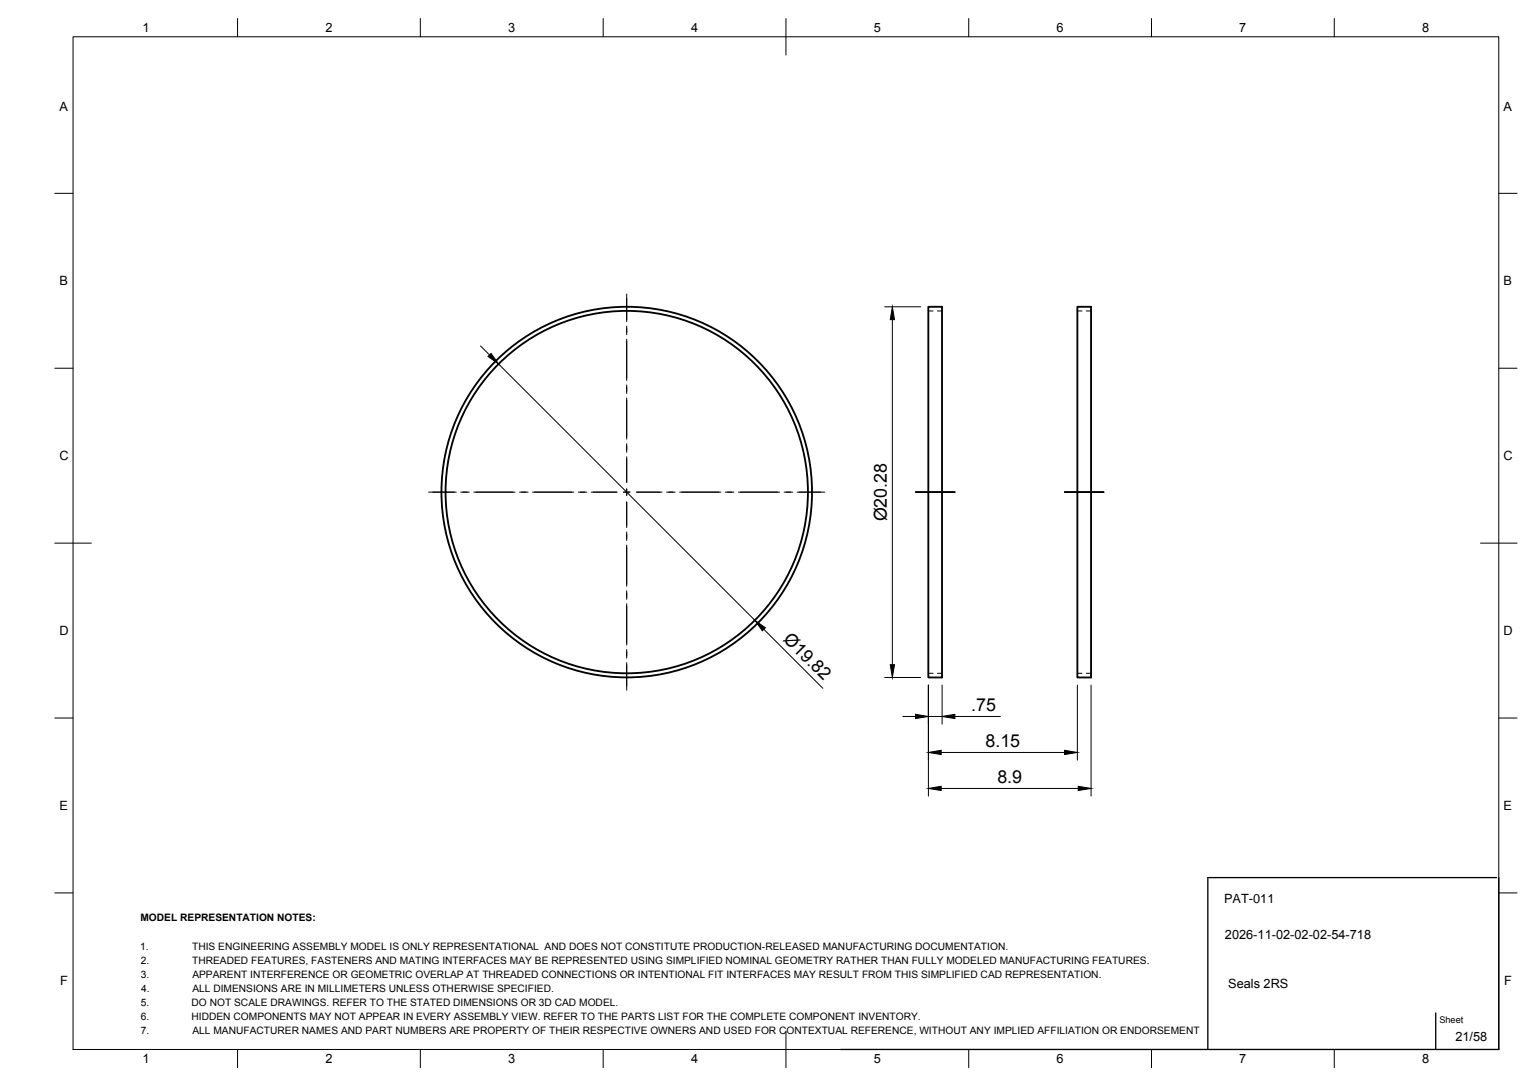
ISO-10303-21;
HEADER;
/* Generated by software containing ST-Developer
 * from STEP Tools, Inc. (www.steptools.com) 
 */

FILE_DESCRIPTION(
/* description */ ('Belt tension measurement rig'),
/* implementation_level */ '2;1');

FILE_NAME(
/* name */ 'Seals 2RS.step',
/* time_stamp */ '2026-10-28T03:24:44-07:00',
/* author */ (''),
/* organization */ (''),
/* preprocessor_version */ 'ST-DEVELOPER v20.2',
/* originating_system */ 'Autodesk Translation Framework v15.17.0.0',
/* authorisation */ '');

FILE_SCHEMA (('AUTOMOTIVE_DESIGN { 1 0 10303 214 3 1 1 }'));
ENDSEC;

DATA;
#10=MECHANICAL_DESIGN_GEOMETRIC_PRESENTATION_REPRESENTATION('',(#717,#718),#23587);
#600=SHAPE_REPRESENTATION_RELATIONSHIP('SRR','None',#23846,#655);
#655=ADVANCED_BREP_SHAPE_REPRESENTATION('',(#787,#788),#23544);
#717=STYLED_ITEM('',(#24211),#787);
#718=STYLED_ITEM('',(#24211),#788);
#787=MANIFOLD_SOLID_BREP('Body1',#12222);
#788=MANIFOLD_SOLID_BREP('Body2',#12223);
#912=FACE_BOUND('',#2360,.T.);
#913=FACE_BOUND('',#2363,.T.);
#914=FACE_BOUND('',#2366,.T.);
#915=FACE_BOUND('',#2369,.T.);
#1151=PLANE('',#13334);
#1152=PLANE('',#13339);
#1153=PLANE('',#13342);
#1154=PLANE('',#13347);
#1572=FACE_OUTER_BOUND('',#2359,.T.);
#1573=FACE_OUTER_BOUND('',#2361,.T.);
#1574=FACE_OUTER_BOUND('',#2362,.T.);
#1575=FACE_OUTER_BOUND('',#2364,.T.);
#1576=FACE_OUTER_BOUND('',#2365,.T.);
#1577=FACE_OUTER_BOUND('',#2367,.T.);
#1578=FACE_OUTER_BOUND('',#2368,.T.);
#1579=FACE_OUTER_BOUND('',#2370,.T.);
#2359=EDGE_LOOP('',(#8872));
#2360=EDGE_LOOP('',(#8873));
#2361=EDGE_LOOP('',(#8874,#8875,#8876,#8877));
#2362=EDGE_LOOP('',(#8878));
#2363=EDGE_LOOP('',(#8879));
#2364=EDGE_LOOP('',(#8880,#8881,#8882,#8883));
#2365=EDGE_LOOP('',(#8884));
#2366=EDGE_LOOP('',(#8885));
#2367=EDGE_LOOP('',(#8886,#8887,#8888,#8889));
#2368=EDGE_LOOP('',(#8890));
#2369=EDGE_LOOP('',(#8891));
#2370=EDGE_LOOP('',(#8892,#8893,#8894,#8895));
#3197=LINE('',#19995,#3948);
#3198=LINE('',#20000,#3949);
#3199=LINE('',#20009,#3950);
#3200=LINE('',#20014,#3951);
#3948=VECTOR('',#15672,1.013815);
#3949=VECTOR('',#15679,0.991185);
#3950=VECTOR('',#15690,1.013815);
#3951=VECTOR('',#15697,0.991185);
#4686=CIRCLE('',#13335,1.013815);
#4687=CIRCLE('',#13336,0.991185);
#4688=CIRCLE('',#13338,1.013815);
#4689=CIRCLE('',#13340,0.991185);
#4690=CIRCLE('',#13343,1.013815);
#4691=CIRCLE('',#13344,0.991185);
#4692=CIRCLE('',#13346,1.013815);
#4693=CIRCLE('',#13348,0.991185);
#5556=VERTEX_POINT('',#19988);
#5557=VERTEX_POINT('',#19990);
#5558=VERTEX_POINT('',#19993);
#5559=VERTEX_POINT('',#19997);
#5560=VERTEX_POINT('',#20002);
#5561=VERTEX_POINT('',#20004);
#5562=VERTEX_POINT('',#20007);
#5563=VERTEX_POINT('',#20011);
#6795=EDGE_CURVE('',#5556,#5556,#4686,.T.);
#6796=EDGE_CURVE('',#5557,#5557,#4687,.T.);
#6797=EDGE_CURVE('',#5558,#5558,#4688,.T.);
#6798=EDGE_CURVE('',#5558,#5556,#3197,.T.);
#6799=EDGE_CURVE('',#5559,#5559,#4689,.T.);
#6800=EDGE_CURVE('',#5559,#5557,#3198,.T.);
#6801=EDGE_CURVE('',#5560,#5560,#4690,.T.);
#6802=EDGE_CURVE('',#5561,#5561,#4691,.T.);
#6803=EDGE_CURVE('',#5562,#5562,#4692,.T.);
#6804=EDGE_CURVE('',#5562,#5560,#3199,.T.);
#6805=EDGE_CURVE('',#5563,#5563,#4693,.T.);
#6806=EDGE_CURVE('',#5563,#5561,#3200,.T.);
#8872=ORIENTED_EDGE('',*,*,#6795,.F.);
#8873=ORIENTED_EDGE('',*,*,#6796,.T.);
#8874=ORIENTED_EDGE('',*,*,#6797,.F.);
#8875=ORIENTED_EDGE('',*,*,#6798,.T.);
#8876=ORIENTED_EDGE('',*,*,#6795,.T.);
#8877=ORIENTED_EDGE('',*,*,#6798,.F.);
#8878=ORIENTED_EDGE('',*,*,#6797,.T.);
#8879=ORIENTED_EDGE('',*,*,#6799,.F.);
#8880=ORIENTED_EDGE('',*,*,#6799,.T.);
#8881=ORIENTED_EDGE('',*,*,#6800,.T.);
#8882=ORIENTED_EDGE('',*,*,#6796,.F.);
#8883=ORIENTED_EDGE('',*,*,#6800,.F.);
#8884=ORIENTED_EDGE('',*,*,#6801,.F.);
#8885=ORIENTED_EDGE('',*,*,#6802,.T.);
#8886=ORIENTED_EDGE('',*,*,#6803,.F.);
#8887=ORIENTED_EDGE('',*,*,#6804,.T.);
#8888=ORIENTED_EDGE('',*,*,#6801,.T.);
#8889=ORIENTED_EDGE('',*,*,#6804,.F.);
#8890=ORIENTED_EDGE('',*,*,#6803,.T.);
#8891=ORIENTED_EDGE('',*,*,#6805,.F.);
#8892=ORIENTED_EDGE('',*,*,#6805,.T.);
#8893=ORIENTED_EDGE('',*,*,#6806,.T.);
#8894=ORIENTED_EDGE('',*,*,#6802,.F.);
#8895=ORIENTED_EDGE('',*,*,#6806,.F.);
#11242=CYLINDRICAL_SURFACE('',#13337,1.013815);
#11243=CYLINDRICAL_SURFACE('',#13341,0.991185);
#11244=CYLINDRICAL_SURFACE('',#13345,1.013815);
#11245=CYLINDRICAL_SURFACE('',#13349,0.991185);
#11713=ADVANCED_FACE('',(#1572,#912),#1151,.T.);
#11714=ADVANCED_FACE('',(#1573),#11242,.T.);
#11715=ADVANCED_FACE('',(#1574,#913),#1152,.T.);
#11716=ADVANCED_FACE('',(#1575),#11243,.F.);
#11717=ADVANCED_FACE('',(#1576,#914),#1153,.T.);
#11718=ADVANCED_FACE('',(#1577),#11244,.T.);
#11719=ADVANCED_FACE('',(#1578,#915),#1154,.T.);
#11720=ADVANCED_FACE('',(#1579),#11245,.F.);
#12222=CLOSED_SHELL('',(#11713,#11714,#11715,#11716));
#12223=CLOSED_SHELL('',(#11717,#11718,#11719,#11720));
#13333=AXIS2_PLACEMENT_3D('',#19986,#15660,#15661);
#13334=AXIS2_PLACEMENT_3D('',#19987,#15662,#15663);
#13335=AXIS2_PLACEMENT_3D('',#19989,#15664,#15665);
#13336=AXIS2_PLACEMENT_3D('',#19991,#15666,#15667);
#13337=AXIS2_PLACEMENT_3D('',#19992,#15668,#15669);
#13338=AXIS2_PLACEMENT_3D('',#19994,#15670,#15671);
#13339=AXIS2_PLACEMENT_3D('',#19996,#15673,#15674);
#13340=AXIS2_PLACEMENT_3D('',#19998,#15675,#15676);
#13341=AXIS2_PLACEMENT_3D('',#19999,#15677,#15678);
#13342=AXIS2_PLACEMENT_3D('',#20001,#15680,#15681);
#13343=AXIS2_PLACEMENT_3D('',#20003,#15682,#15683);
#13344=AXIS2_PLACEMENT_3D('',#20005,#15684,#15685);
#13345=AXIS2_PLACEMENT_3D('',#20006,#15686,#15687);
#13346=AXIS2_PLACEMENT_3D('',#20008,#15688,#15689);
#13347=AXIS2_PLACEMENT_3D('',#20010,#15691,#15692);
#13348=AXIS2_PLACEMENT_3D('',#20012,#15693,#15694);
#13349=AXIS2_PLACEMENT_3D('',#20013,#15695,#15696);
#15660=DIRECTION('axis',(0.,0.,1.));
#15661=DIRECTION('refdir',(1.,0.,0.));
#15662=DIRECTION('center_axis',(0.,1.,0.));
#15663=DIRECTION('ref_axis',(0.,0.,1.));
#15664=DIRECTION('center_axis',(0.,-1.,0.));
#15665=DIRECTION('ref_axis',(1.,0.,0.));
#15666=DIRECTION('center_axis',(0.,-1.,0.));
#15667=DIRECTION('ref_axis',(1.,0.,0.));
#15668=DIRECTION('center_axis',(0.,-1.,0.));
#15669=DIRECTION('ref_axis',(1.,0.,0.));
#15670=DIRECTION('center_axis',(0.,-1.,0.));
#15671=DIRECTION('ref_axis',(1.,0.,0.));
#15672=DIRECTION('',(0.,1.,0.));
#15673=DIRECTION('center_axis',(0.,-1.,0.));
#15674=DIRECTION('ref_axis',(0.,0.,-1.));
#15675=DIRECTION('center_axis',(0.,-1.,0.));
#15676=DIRECTION('ref_axis',(1.,0.,0.));
#15677=DIRECTION('center_axis',(0.,-1.,0.));
#15678=DIRECTION('ref_axis',(1.,0.,0.));
#15679=DIRECTION('',(0.,1.,0.));
#15680=DIRECTION('center_axis',(0.,1.,0.));
#15681=DIRECTION('ref_axis',(0.,0.,1.));
#15682=DIRECTION('center_axis',(0.,-1.,0.));
#15683=DIRECTION('ref_axis',(1.,0.,0.));
#15684=DIRECTION('center_axis',(0.,-1.,0.));
#15685=DIRECTION('ref_axis',(1.,0.,0.));
#15686=DIRECTION('center_axis',(0.,-1.,0.));
#15687=DIRECTION('ref_axis',(1.,0.,0.));
#15688=DIRECTION('center_axis',(0.,-1.,0.));
#15689=DIRECTION('ref_axis',(1.,0.,0.));
#15690=DIRECTION('',(0.,1.,0.));
#15691=DIRECTION('center_axis',(0.,-1.,0.));
#15692=DIRECTION('ref_axis',(0.,0.,-1.));
#15693=DIRECTION('center_axis',(0.,-1.,0.));
#15694=DIRECTION('ref_axis',(1.,0.,0.));
#15695=DIRECTION('center_axis',(0.,-1.,0.));
#15696=DIRECTION('ref_axis',(1.,0.,0.));
#15697=DIRECTION('',(0.,1.,0.));
#19986=CARTESIAN_POINT('',(0.,0.,0.));
#19987=CARTESIAN_POINT('Origin',(1.013815,0.445,0.));
#19988=CARTESIAN_POINT('',(-1.013815,0.445,-1.24156529467757E-16));
#19989=CARTESIAN_POINT('Origin',(0.,0.445,0.));
#19990=CARTESIAN_POINT('',(-0.991185,0.445,-1.21385153761287E-16));
#19991=CARTESIAN_POINT('Origin',(0.,0.445,0.));
#19992=CARTESIAN_POINT('Origin',(0.,0.4075,0.));
#19993=CARTESIAN_POINT('',(-1.013815,0.37,-1.24156529467757E-16));
#19994=CARTESIAN_POINT('Origin',(0.,0.37,0.));
#19995=CARTESIAN_POINT('',(-1.013815,0.4075,-1.24156529467757E-16));
#19996=CARTESIAN_POINT('Origin',(0.991185,0.37,0.));
#19997=CARTESIAN_POINT('',(-0.991185,0.37,-1.21385153761287E-16));
#19998=CARTESIAN_POINT('Origin',(0.,0.37,0.));
#19999=CARTESIAN_POINT('Origin',(0.,0.4075,0.));
#20000=CARTESIAN_POINT('',(-0.991185,0.4075,-1.21385153761287E-16));
#20001=CARTESIAN_POINT('Origin',(1.013815,-0.37,0.));
#20002=CARTESIAN_POINT('',(-1.013815,-0.37,-1.24156529467757E-16));
#20003=CARTESIAN_POINT('Origin',(0.,-0.37,0.));
#20004=CARTESIAN_POINT('',(-0.991185,-0.37,-1.21385153761287E-16));
#20005=CARTESIAN_POINT('Origin',(0.,-0.37,0.));
#20006=CARTESIAN_POINT('Origin',(0.,-0.4075,0.));
#20007=CARTESIAN_POINT('',(-1.013815,-0.445,-1.24156529467757E-16));
#20008=CARTESIAN_POINT('Origin',(0.,-0.445,0.));
#20009=CARTESIAN_POINT('',(-1.013815,-0.4075,-1.24156529467757E-16));
#20010=CARTESIAN_POINT('Origin',(0.991185,-0.445,0.));
#20011=CARTESIAN_POINT('',(-0.991185,-0.445,-1.21385153761287E-16));
#20012=CARTESIAN_POINT('Origin',(0.,-0.445,0.));
#20013=CARTESIAN_POINT('Origin',(0.,-0.4075,0.));
#20014=CARTESIAN_POINT('',(-0.991185,-0.4075,-1.21385153761287E-16));
#23479=UNCERTAINTY_MEASURE_WITH_UNIT(LENGTH_MEASURE(0.001),#23588,
'DISTANCE_ACCURACY_VALUE',
'Maximum model space distance between geometric entities at asserted c
onnectivities');
#23522=UNCERTAINTY_MEASURE_WITH_UNIT(LENGTH_MEASURE(0.001),#23588,
'DISTANCE_ACCURACY_VALUE',
'Maximum model space distance between geometric entities at asserted c
onnectivities');
#23544=(
GEOMETRIC_REPRESENTATION_CONTEXT(3)
GLOBAL_UNCERTAINTY_ASSIGNED_CONTEXT((#23479))
GLOBAL_UNIT_ASSIGNED_CONTEXT((#23588,#23590,#23591))
REPRESENTATION_CONTEXT('','3D')
);
#23587=(
GEOMETRIC_REPRESENTATION_CONTEXT(3)
GLOBAL_UNCERTAINTY_ASSIGNED_CONTEXT((#23522))
GLOBAL_UNIT_ASSIGNED_CONTEXT((#23588,#23590,#23591))
REPRESENTATION_CONTEXT('','3D')
);
#23588=(
LENGTH_UNIT()
NAMED_UNIT(*)
SI_UNIT(.CENTI.,.METRE.)
);
#23590=(
NAMED_UNIT(*)
PLANE_ANGLE_UNIT()
SI_UNIT($,.RADIAN.)
);
#23591=(
NAMED_UNIT(*)
SI_UNIT($,.STERADIAN.)
SOLID_ANGLE_UNIT()
);
#23613=SHAPE_DEFINITION_REPRESENTATION(#23677,#23846);
#23677=PRODUCT_DEFINITION_SHAPE('',$,#23911);
#23846=SHAPE_REPRESENTATION('',(#13333),#23544);
#23889=PRODUCT_DEFINITION_CONTEXT('part definition',#24083,'design');
#23911=PRODUCT_DEFINITION('Seals 2RS','Seals 2RS',#23975,#23889);
#23975=PRODUCT_DEFINITION_FORMATION('',$,#24106);
#24083=APPLICATION_CONTEXT(
'Core Data for Automotive Mechanical Design Process');
#24084=PRODUCT_CONTEXT('part definition',#24083,'mechanical');
#24106=PRODUCT('Seals 2RS','Seals 2RS','Seals 2RS',(#24084));
#24205=COLOUR_RGB('Grey',0.48,0.52,0.57);
#24206=FILL_AREA_STYLE_COLOUR('',#24205);
#24207=FILL_AREA_STYLE('',(#24206));
#24208=SURFACE_STYLE_FILL_AREA(#24207);
#24209=SURFACE_SIDE_STYLE('',(#24208));
#24210=SURFACE_STYLE_USAGE(.BOTH.,#24209);
#24211=PRESENTATION_STYLE_ASSIGNMENT((#24210));
ENDSEC;
END-ISO-10303-21;
